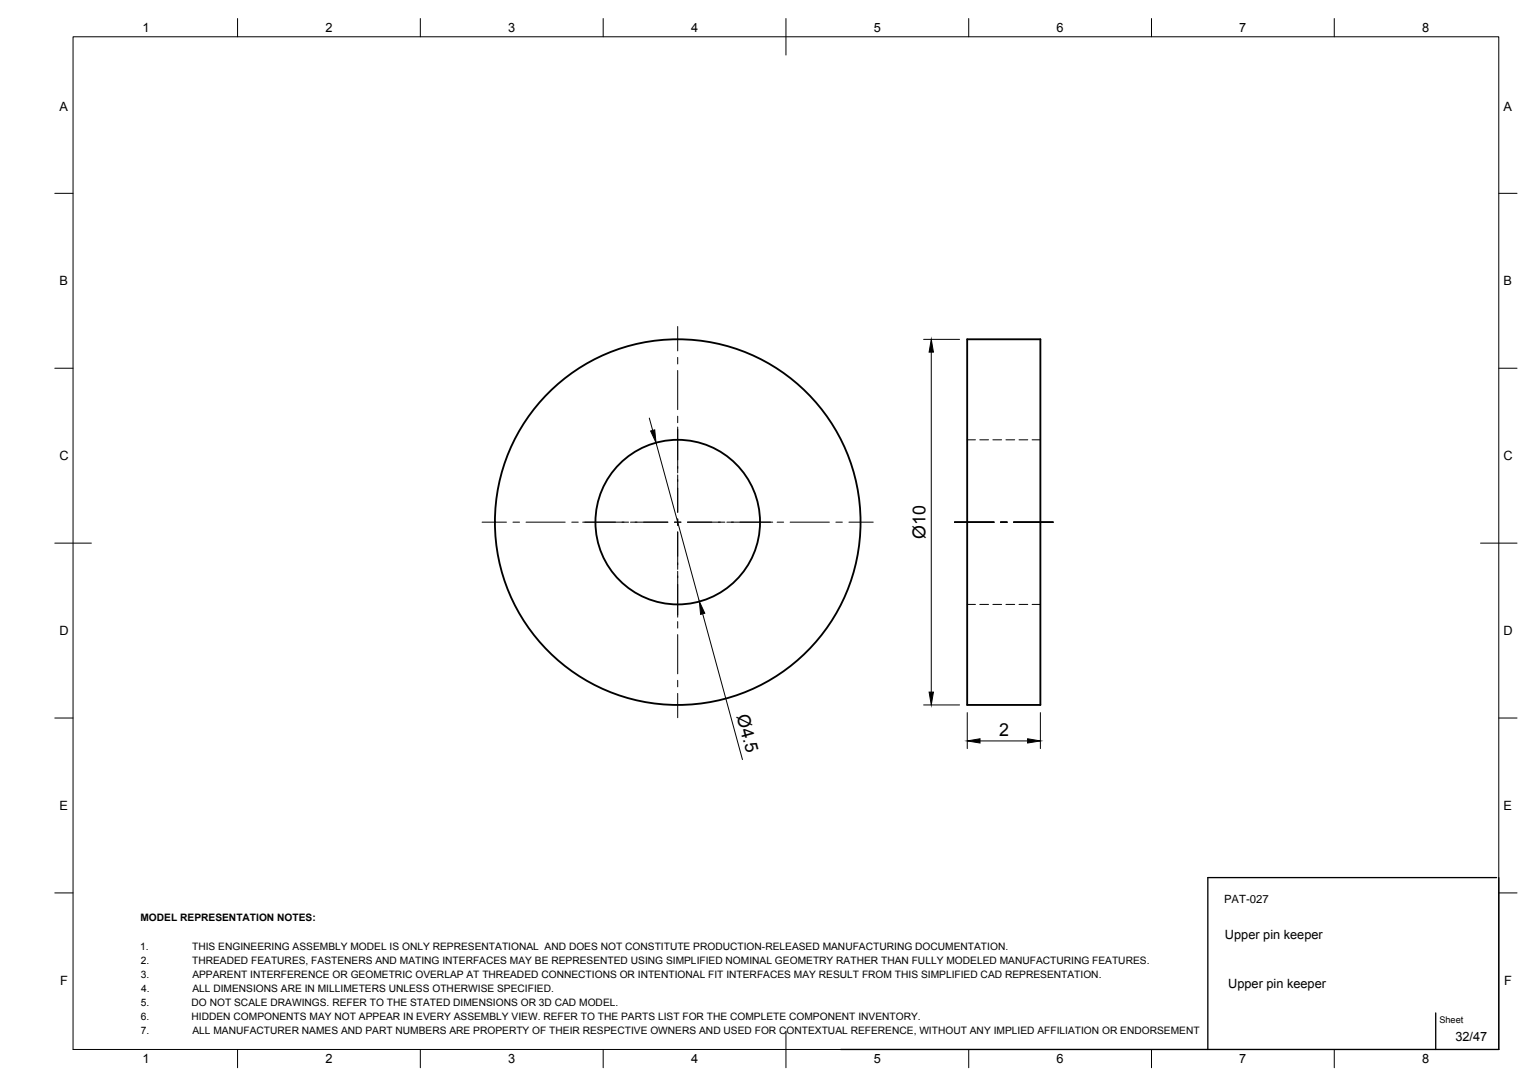
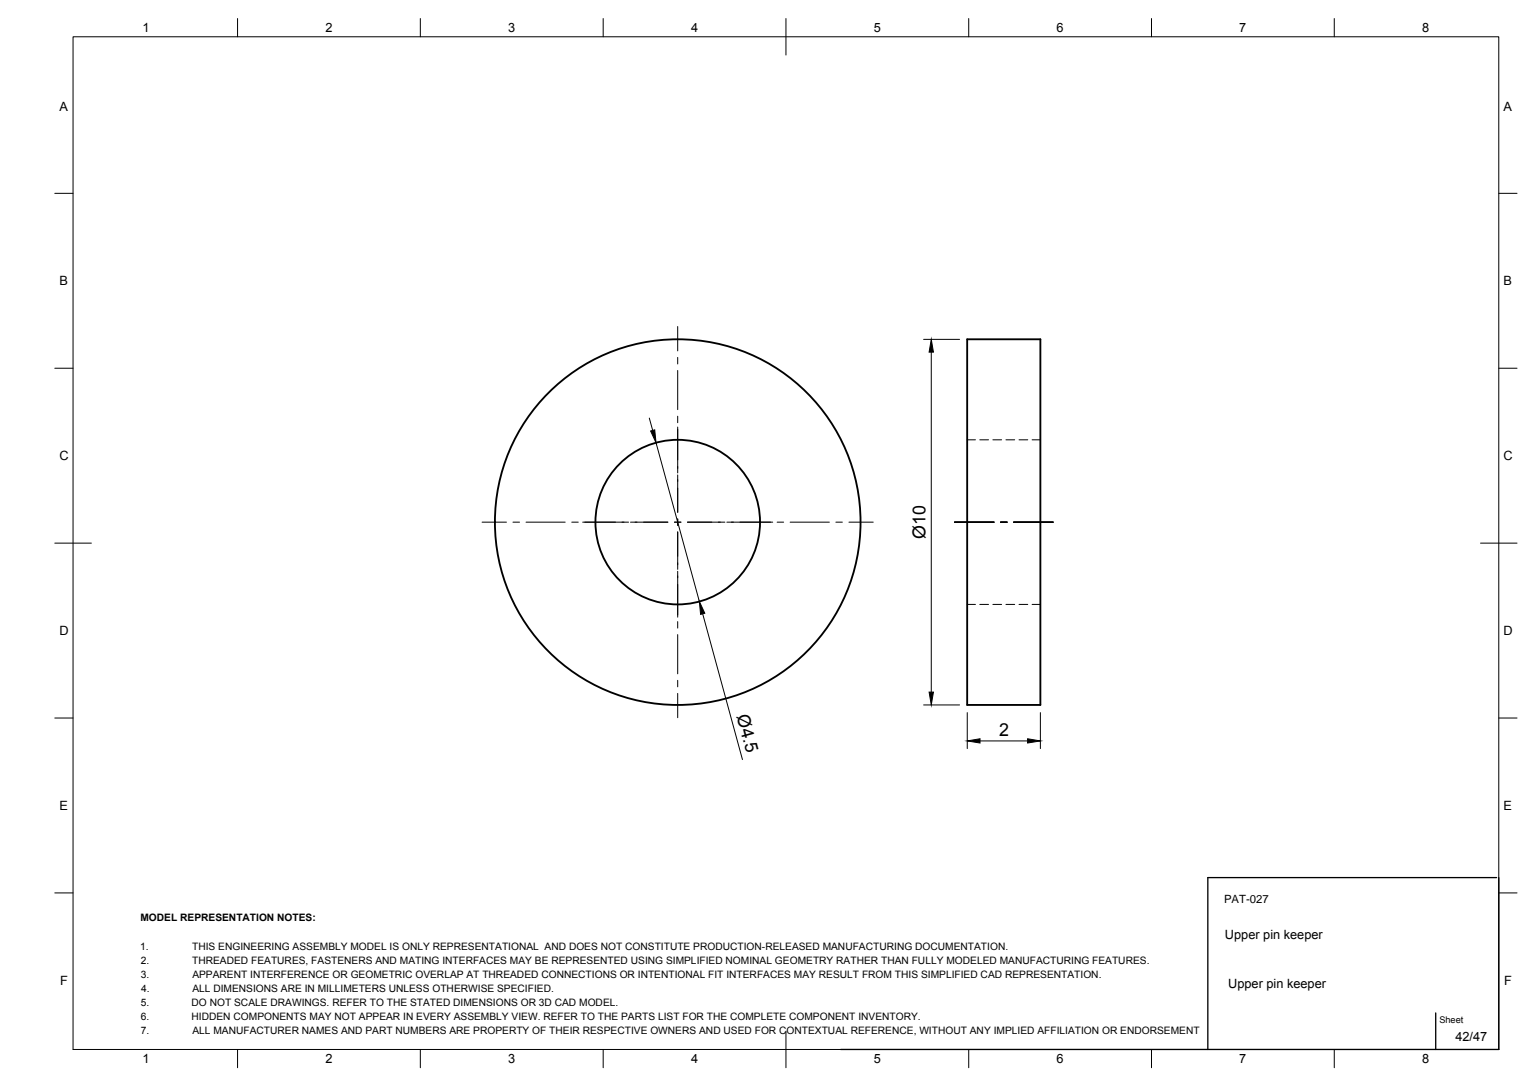
ISO-10303-21;
HEADER;
/* Generated by software containing ST-Developer
 * from STEP Tools, Inc. (www.steptools.com) 
 */

FILE_DESCRIPTION(
/* description */ ('Crank-driven oscillating fan base (mechanism only)'),

/* implementation_level */ '2;1');

FILE_NAME(
/* name */ 'Upper pin keeper.step',
/* time_stamp */ '2026-10-28T03:25:00-07:00',
/* author */ (''),
/* organization */ (''),
/* preprocessor_version */ 'ST-DEVELOPER v20.2',
/* originating_system */ 'Autodesk Translation Framework v15.17.0.0',
/* authorisation */ '');

FILE_SCHEMA (('AUTOMOTIVE_DESIGN { 1 0 10303 214 3 1 1 }'));
ENDSEC;

DATA;
#10=MECHANICAL_DESIGN_GEOMETRIC_PRESENTATION_REPRESENTATION('',(#469),#11916);
#381=SHAPE_REPRESENTATION_RELATIONSHIP('SRR','None',#12107,#421);
#421=ADVANCED_BREP_SHAPE_REPRESENTATION('',(#516),#11898);
#469=STYLED_ITEM('',(#12375),#516);
#516=MANIFOLD_SOLID_BREP('Body1',#6100);
#646=FACE_BOUND('',#1619,.T.);
#647=FACE_BOUND('',#1621,.T.);
#804=PLANE('',#7105);
#805=PLANE('',#7106);
#1125=FACE_OUTER_BOUND('',#1616,.T.);
#1126=FACE_OUTER_BOUND('',#1617,.T.);
#1127=FACE_OUTER_BOUND('',#1618,.T.);
#1128=FACE_OUTER_BOUND('',#1620,.T.);
#1616=EDGE_LOOP('',(#5036,#5037,#5038,#5039));
#1617=EDGE_LOOP('',(#5040,#5041,#5042,#5043));
#1618=EDGE_LOOP('',(#5044));
#1619=EDGE_LOOP('',(#5045));
#1620=EDGE_LOOP('',(#5046));
#1621=EDGE_LOOP('',(#5047));
#1979=LINE('',#11130,#2312);
#1980=LINE('',#11136,#2313);
#2312=VECTOR('',#8676,0.225);
#2313=VECTOR('',#8683,0.5);
#2731=CIRCLE('',#7100,0.225);
#2732=CIRCLE('',#7101,0.225);
#2733=CIRCLE('',#7103,0.5);
#2734=CIRCLE('',#7104,0.5);
#3162=VERTEX_POINT('',#11127);
#3163=VERTEX_POINT('',#11129);
#3164=VERTEX_POINT('',#11133);
#3165=VERTEX_POINT('',#11135);
#3813=EDGE_CURVE('',#3162,#3162,#2731,.T.);
#3814=EDGE_CURVE('',#3162,#3163,#1979,.T.);
#3815=EDGE_CURVE('',#3163,#3163,#2732,.T.);
#3816=EDGE_CURVE('',#3164,#3164,#2733,.T.);
#3817=EDGE_CURVE('',#3164,#3165,#1980,.T.);
#3818=EDGE_CURVE('',#3165,#3165,#2734,.T.);
#5036=ORIENTED_EDGE('',*,*,#3813,.F.);
#5037=ORIENTED_EDGE('',*,*,#3814,.T.);
#5038=ORIENTED_EDGE('',*,*,#3815,.T.);
#5039=ORIENTED_EDGE('',*,*,#3814,.F.);
#5040=ORIENTED_EDGE('',*,*,#3816,.F.);
#5041=ORIENTED_EDGE('',*,*,#3817,.T.);
#5042=ORIENTED_EDGE('',*,*,#3818,.T.);
#5043=ORIENTED_EDGE('',*,*,#3817,.F.);
#5044=ORIENTED_EDGE('',*,*,#3816,.T.);
#5045=ORIENTED_EDGE('',*,*,#3813,.T.);
#5046=ORIENTED_EDGE('',*,*,#3818,.F.);
#5047=ORIENTED_EDGE('',*,*,#3815,.F.);
#5648=CYLINDRICAL_SURFACE('',#7099,0.225);
#5649=CYLINDRICAL_SURFACE('',#7102,0.5);
#5931=ADVANCED_FACE('',(#1125),#5648,.F.);
#5932=ADVANCED_FACE('',(#1126),#5649,.T.);
#5933=ADVANCED_FACE('',(#1127,#646),#804,.T.);
#5934=ADVANCED_FACE('',(#1128,#647),#805,.F.);
#6100=CLOSED_SHELL('',(#5931,#5932,#5933,#5934));
#7098=AXIS2_PLACEMENT_3D('',#11125,#8670,#8671);
#7099=AXIS2_PLACEMENT_3D('',#11126,#8672,#8673);
#7100=AXIS2_PLACEMENT_3D('',#11128,#8674,#8675);
#7101=AXIS2_PLACEMENT_3D('',#11131,#8677,#8678);
#7102=AXIS2_PLACEMENT_3D('',#11132,#8679,#8680);
#7103=AXIS2_PLACEMENT_3D('',#11134,#8681,#8682);
#7104=AXIS2_PLACEMENT_3D('',#11137,#8684,#8685);
#7105=AXIS2_PLACEMENT_3D('',#11138,#8686,#8687);
#7106=AXIS2_PLACEMENT_3D('',#11139,#8688,#8689);
#8670=DIRECTION('axis',(0.,0.,1.));
#8671=DIRECTION('refdir',(1.,0.,0.));
#8672=DIRECTION('center_axis',(0.,0.,1.));
#8673=DIRECTION('ref_axis',(1.,0.,0.));
#8674=DIRECTION('center_axis',(0.,0.,-1.));
#8675=DIRECTION('ref_axis',(1.,0.,0.));
#8676=DIRECTION('',(0.,0.,-1.));
#8677=DIRECTION('center_axis',(0.,0.,-1.));
#8678=DIRECTION('ref_axis',(1.,0.,0.));
#8679=DIRECTION('center_axis',(0.,0.,1.));
#8680=DIRECTION('ref_axis',(1.,0.,0.));
#8681=DIRECTION('center_axis',(0.,0.,1.));
#8682=DIRECTION('ref_axis',(1.,0.,0.));
#8683=DIRECTION('',(0.,0.,-1.));
#8684=DIRECTION('center_axis',(0.,0.,1.));
#8685=DIRECTION('ref_axis',(1.,0.,0.));
#8686=DIRECTION('center_axis',(0.,0.,1.));
#8687=DIRECTION('ref_axis',(1.,0.,0.));
#8688=DIRECTION('center_axis',(0.,0.,1.));
#8689=DIRECTION('ref_axis',(1.,0.,0.));
#11125=CARTESIAN_POINT('',(0.,0.,0.));
#11126=CARTESIAN_POINT('Origin',(-0.429855350392604,2.61349944954989,9.6));
#11127=CARTESIAN_POINT('',(-0.654855350392604,2.61349944954989,9.8));
#11128=CARTESIAN_POINT('Origin',(-0.429855350392604,2.61349944954989,9.8));
#11129=CARTESIAN_POINT('',(-0.654855350392604,2.61349944954989,9.6));
#11130=CARTESIAN_POINT('',(-0.654855350392604,2.61349944954989,9.6));
#11131=CARTESIAN_POINT('Origin',(-0.429855350392604,2.61349944954989,9.6));
#11132=CARTESIAN_POINT('Origin',(-0.429855350392604,2.61349944954989,9.6));
#11133=CARTESIAN_POINT('',(-0.929855350392604,2.61349944954989,9.8));
#11134=CARTESIAN_POINT('Origin',(-0.429855350392604,2.61349944954989,9.8));
#11135=CARTESIAN_POINT('',(-0.929855350392604,2.61349944954989,9.6));
#11136=CARTESIAN_POINT('',(-0.929855350392604,2.61349944954989,9.6));
#11137=CARTESIAN_POINT('Origin',(-0.429855350392604,2.61349944954989,9.6));
#11138=CARTESIAN_POINT('Origin',(-0.429855350392604,2.61349944954989,9.8));
#11139=CARTESIAN_POINT('Origin',(-0.429855350392604,2.61349944954989,9.6));
#11851=UNCERTAINTY_MEASURE_WITH_UNIT(LENGTH_MEASURE(0.001),#11917,
'DISTANCE_ACCURACY_VALUE',
'Maximum model space distance between geometric entities at asserted c
onnectivities');
#11869=UNCERTAINTY_MEASURE_WITH_UNIT(LENGTH_MEASURE(0.001),#11917,
'DISTANCE_ACCURACY_VALUE',
'Maximum model space distance between geometric entities at asserted c
onnectivities');
#11898=(
GEOMETRIC_REPRESENTATION_CONTEXT(3)
GLOBAL_UNCERTAINTY_ASSIGNED_CONTEXT((#11851))
GLOBAL_UNIT_ASSIGNED_CONTEXT((#11917,#11919,#11920))
REPRESENTATION_CONTEXT('','3D')
);
#11916=(
GEOMETRIC_REPRESENTATION_CONTEXT(3)
GLOBAL_UNCERTAINTY_ASSIGNED_CONTEXT((#11869))
GLOBAL_UNIT_ASSIGNED_CONTEXT((#11917,#11919,#11920))
REPRESENTATION_CONTEXT('','3D')
);
#11917=(
LENGTH_UNIT()
NAMED_UNIT(*)
SI_UNIT(.CENTI.,.METRE.)
);
#11919=(
NAMED_UNIT(*)
PLANE_ANGLE_UNIT()
SI_UNIT($,.RADIAN.)
);
#11920=(
NAMED_UNIT(*)
SI_UNIT($,.STERADIAN.)
SOLID_ANGLE_UNIT()
);
#11949=SHAPE_DEFINITION_REPRESENTATION(#12000,#12107);
#12000=PRODUCT_DEFINITION_SHAPE('',$,#12154);
#12107=SHAPE_REPRESENTATION('',(#7098),#11898);
#12125=PRODUCT_DEFINITION_CONTEXT('part definition',#12265,'design');
#12154=PRODUCT_DEFINITION('Upper pin keeper','Upper pin keeper',#12200,
#12125);
#12200=PRODUCT_DEFINITION_FORMATION('',$,#12295);
#12265=APPLICATION_CONTEXT(
'Core Data for Automotive Mechanical Design Process');
#12266=PRODUCT_CONTEXT('part definition',#12265,'mechanical');
#12295=PRODUCT('Upper pin keeper','Upper pin keeper','Upper pin keeper',
(#12266));
#12369=COLOUR_RGB('Grey',0.48,0.52,0.57);
#12370=FILL_AREA_STYLE_COLOUR('',#12369);
#12371=FILL_AREA_STYLE('',(#12370));
#12372=SURFACE_STYLE_FILL_AREA(#12371);
#12373=SURFACE_SIDE_STYLE('',(#12372));
#12374=SURFACE_STYLE_USAGE(.BOTH.,#12373);
#12375=PRESENTATION_STYLE_ASSIGNMENT((#12374));
ENDSEC;
END-ISO-10303-21;
